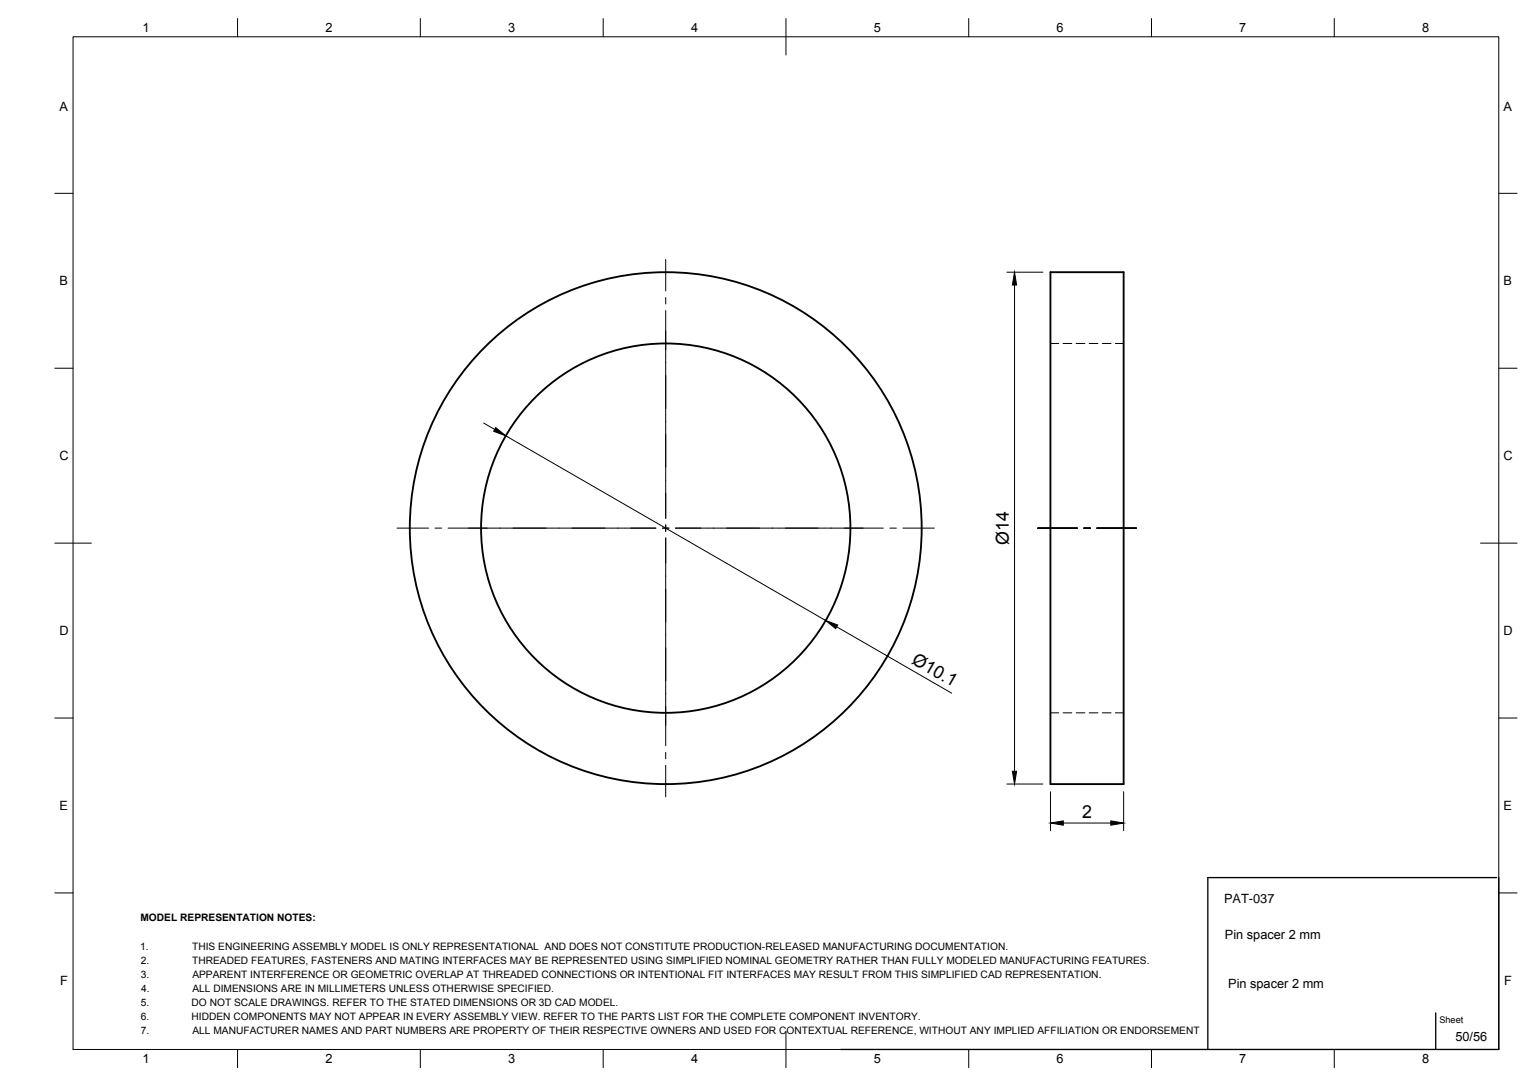
ISO-10303-21;
HEADER;
/* Generated by software containing ST-Developer
 * from STEP Tools, Inc. (www.steptools.com) 
 */

FILE_DESCRIPTION(
/* description */ ('Flywheel Crank-Slider'),
/* implementation_level */ '2;1');

FILE_NAME(
/* name */ 'Pin spacer 2 mm.step',
/* time_stamp */ '2026-10-28T03:23:13-07:00',
/* author */ (''),
/* organization */ (''),
/* preprocessor_version */ 'ST-DEVELOPER v20.2',
/* originating_system */ 'Autodesk Translation Framework v15.17.0.0',
/* authorisation */ '');

FILE_SCHEMA (('AUTOMOTIVE_DESIGN { 1 0 10303 214 3 1 1 }'));
ENDSEC;

DATA;
#10=MECHANICAL_DESIGN_GEOMETRIC_PRESENTATION_REPRESENTATION('',(#723),#17322);
#610=SHAPE_REPRESENTATION_RELATIONSHIP('SRR','None',#17611,#662);
#662=ADVANCED_BREP_SHAPE_REPRESENTATION('',(#780),#17315);
#723=STYLED_ITEM('',(#17931),#780);
#780=MANIFOLD_SOLID_BREP('Body1',#9105);
#993=FACE_BOUND('',#2548,.T.);
#994=FACE_BOUND('',#2550,.T.);
#1286=PLANE('',#10639);
#1287=PLANE('',#10640);
#1802=FACE_OUTER_BOUND('',#2545,.T.);
#1803=FACE_OUTER_BOUND('',#2546,.T.);
#1804=FACE_OUTER_BOUND('',#2547,.T.);
#1805=FACE_OUTER_BOUND('',#2549,.T.);
#2545=EDGE_LOOP('',(#8138,#8139,#8140,#8141));
#2546=EDGE_LOOP('',(#8142,#8143,#8144,#8145));
#2547=EDGE_LOOP('',(#8146));
#2548=EDGE_LOOP('',(#8147));
#2549=EDGE_LOOP('',(#8148));
#2550=EDGE_LOOP('',(#8149));
#3172=LINE('',#16890,#3783);
#3173=LINE('',#16896,#3784);
#3783=VECTOR('',#13286,0.505000000000001);
#3784=VECTOR('',#13293,0.699999999999999);
#4236=CIRCLE('',#10634,0.505000000000001);
#4237=CIRCLE('',#10635,0.505000000000001);
#4238=CIRCLE('',#10637,0.699999999999999);
#4239=CIRCLE('',#10638,0.699999999999999);
#4955=VERTEX_POINT('',#16887);
#4956=VERTEX_POINT('',#16889);
#4957=VERTEX_POINT('',#16893);
#4958=VERTEX_POINT('',#16895);
#6026=EDGE_CURVE('',#4955,#4955,#4236,.T.);
#6027=EDGE_CURVE('',#4955,#4956,#3172,.T.);
#6028=EDGE_CURVE('',#4956,#4956,#4237,.T.);
#6029=EDGE_CURVE('',#4957,#4957,#4238,.T.);
#6030=EDGE_CURVE('',#4957,#4958,#3173,.T.);
#6031=EDGE_CURVE('',#4958,#4958,#4239,.T.);
#8138=ORIENTED_EDGE('',*,*,#6026,.F.);
#8139=ORIENTED_EDGE('',*,*,#6027,.T.);
#8140=ORIENTED_EDGE('',*,*,#6028,.T.);
#8141=ORIENTED_EDGE('',*,*,#6027,.F.);
#8142=ORIENTED_EDGE('',*,*,#6029,.F.);
#8143=ORIENTED_EDGE('',*,*,#6030,.T.);
#8144=ORIENTED_EDGE('',*,*,#6031,.T.);
#8145=ORIENTED_EDGE('',*,*,#6030,.F.);
#8146=ORIENTED_EDGE('',*,*,#6029,.T.);
#8147=ORIENTED_EDGE('',*,*,#6026,.T.);
#8148=ORIENTED_EDGE('',*,*,#6031,.F.);
#8149=ORIENTED_EDGE('',*,*,#6028,.F.);
#8495=CYLINDRICAL_SURFACE('',#10633,0.505000000000001);
#8496=CYLINDRICAL_SURFACE('',#10636,0.699999999999999);
#8993=ADVANCED_FACE('',(#1802),#8495,.F.);
#8994=ADVANCED_FACE('',(#1803),#8496,.T.);
#8995=ADVANCED_FACE('',(#1804,#993),#1286,.T.);
#8996=ADVANCED_FACE('',(#1805,#994),#1287,.F.);
#9105=CLOSED_SHELL('',(#8993,#8994,#8995,#8996));
#10632=AXIS2_PLACEMENT_3D('',#16885,#13280,#13281);
#10633=AXIS2_PLACEMENT_3D('',#16886,#13282,#13283);
#10634=AXIS2_PLACEMENT_3D('',#16888,#13284,#13285);
#10635=AXIS2_PLACEMENT_3D('',#16891,#13287,#13288);
#10636=AXIS2_PLACEMENT_3D('',#16892,#13289,#13290);
#10637=AXIS2_PLACEMENT_3D('',#16894,#13291,#13292);
#10638=AXIS2_PLACEMENT_3D('',#16897,#13294,#13295);
#10639=AXIS2_PLACEMENT_3D('',#16898,#13296,#13297);
#10640=AXIS2_PLACEMENT_3D('',#16899,#13298,#13299);
#13280=DIRECTION('axis',(0.,0.,1.));
#13281=DIRECTION('refdir',(1.,0.,0.));
#13282=DIRECTION('center_axis',(0.,1.,0.));
#13283=DIRECTION('ref_axis',(1.,0.,0.));
#13284=DIRECTION('center_axis',(0.,-1.,0.));
#13285=DIRECTION('ref_axis',(1.,0.,0.));
#13286=DIRECTION('',(0.,-1.,0.));
#13287=DIRECTION('center_axis',(0.,-1.,0.));
#13288=DIRECTION('ref_axis',(1.,0.,0.));
#13289=DIRECTION('center_axis',(0.,1.,0.));
#13290=DIRECTION('ref_axis',(1.,0.,0.));
#13291=DIRECTION('center_axis',(0.,1.,0.));
#13292=DIRECTION('ref_axis',(1.,0.,0.));
#13293=DIRECTION('',(0.,-1.,0.));
#13294=DIRECTION('center_axis',(0.,1.,0.));
#13295=DIRECTION('ref_axis',(1.,0.,0.));
#13296=DIRECTION('center_axis',(0.,1.,0.));
#13297=DIRECTION('ref_axis',(1.,0.,0.));
#13298=DIRECTION('center_axis',(0.,1.,0.));
#13299=DIRECTION('ref_axis',(1.,0.,0.));
#16885=CARTESIAN_POINT('',(0.,0.,0.));
#16886=CARTESIAN_POINT('Origin',(12.,2.3,10.));
#16887=CARTESIAN_POINT('',(11.495,2.5,10.));
#16888=CARTESIAN_POINT('Origin',(12.,2.5,10.));
#16889=CARTESIAN_POINT('',(11.495,2.3,10.));
#16890=CARTESIAN_POINT('',(11.495,2.3,10.));
#16891=CARTESIAN_POINT('Origin',(12.,2.3,10.));
#16892=CARTESIAN_POINT('Origin',(12.,2.3,10.));
#16893=CARTESIAN_POINT('',(11.3,2.5,10.));
#16894=CARTESIAN_POINT('Origin',(12.,2.5,10.));
#16895=CARTESIAN_POINT('',(11.3,2.3,10.));
#16896=CARTESIAN_POINT('',(11.3,2.3,10.));
#16897=CARTESIAN_POINT('Origin',(12.,2.3,10.));
#16898=CARTESIAN_POINT('Origin',(12.,2.5,10.));
#16899=CARTESIAN_POINT('Origin',(12.,2.3,10.));
#17254=UNCERTAINTY_MEASURE_WITH_UNIT(LENGTH_MEASURE(0.001),#17323,
'DISTANCE_ACCURACY_VALUE',
'Maximum model space distance between geometric entities at asserted c
onnectivities');
#17261=UNCERTAINTY_MEASURE_WITH_UNIT(LENGTH_MEASURE(0.001),#17323,
'DISTANCE_ACCURACY_VALUE',
'Maximum model space distance between geometric entities at asserted c
onnectivities');
#17315=(
GEOMETRIC_REPRESENTATION_CONTEXT(3)
GLOBAL_UNCERTAINTY_ASSIGNED_CONTEXT((#17254))
GLOBAL_UNIT_ASSIGNED_CONTEXT((#17323,#17325,#17326))
REPRESENTATION_CONTEXT('','3D')
);
#17322=(
GEOMETRIC_REPRESENTATION_CONTEXT(3)
GLOBAL_UNCERTAINTY_ASSIGNED_CONTEXT((#17261))
GLOBAL_UNIT_ASSIGNED_CONTEXT((#17323,#17325,#17326))
REPRESENTATION_CONTEXT('','3D')
);
#17323=(
LENGTH_UNIT()
NAMED_UNIT(*)
SI_UNIT(.CENTI.,.METRE.)
);
#17325=(
NAMED_UNIT(*)
PLANE_ANGLE_UNIT()
SI_UNIT($,.RADIAN.)
);
#17326=(
NAMED_UNIT(*)
SI_UNIT($,.STERADIAN.)
SOLID_ANGLE_UNIT()
);
#17380=SHAPE_DEFINITION_REPRESENTATION(#17454,#17611);
#17454=PRODUCT_DEFINITION_SHAPE('',$,#17672);
#17611=SHAPE_REPRESENTATION('',(#10632),#17315);
#17618=PRODUCT_DEFINITION_CONTEXT('part definition',#17800,'design');
#17672=PRODUCT_DEFINITION('Pin spacer 2 mm','Pin spacer 2 mm',#17732,#17618);
#17732=PRODUCT_DEFINITION_FORMATION('',$,#17855);
#17800=APPLICATION_CONTEXT(
'Core Data for Automotive Mechanical Design Process');
#17801=PRODUCT_CONTEXT('part definition',#17800,'mechanical');
#17855=PRODUCT('Pin spacer 2 mm','Pin spacer 2 mm','Pin spacer 2 mm',(#17801));
#17925=COLOUR_RGB('Grey',0.48,0.52,0.57);
#17926=FILL_AREA_STYLE_COLOUR('',#17925);
#17927=FILL_AREA_STYLE('',(#17926));
#17928=SURFACE_STYLE_FILL_AREA(#17927);
#17929=SURFACE_SIDE_STYLE('',(#17928));
#17930=SURFACE_STYLE_USAGE(.BOTH.,#17929);
#17931=PRESENTATION_STYLE_ASSIGNMENT((#17930));
ENDSEC;
END-ISO-10303-21;
